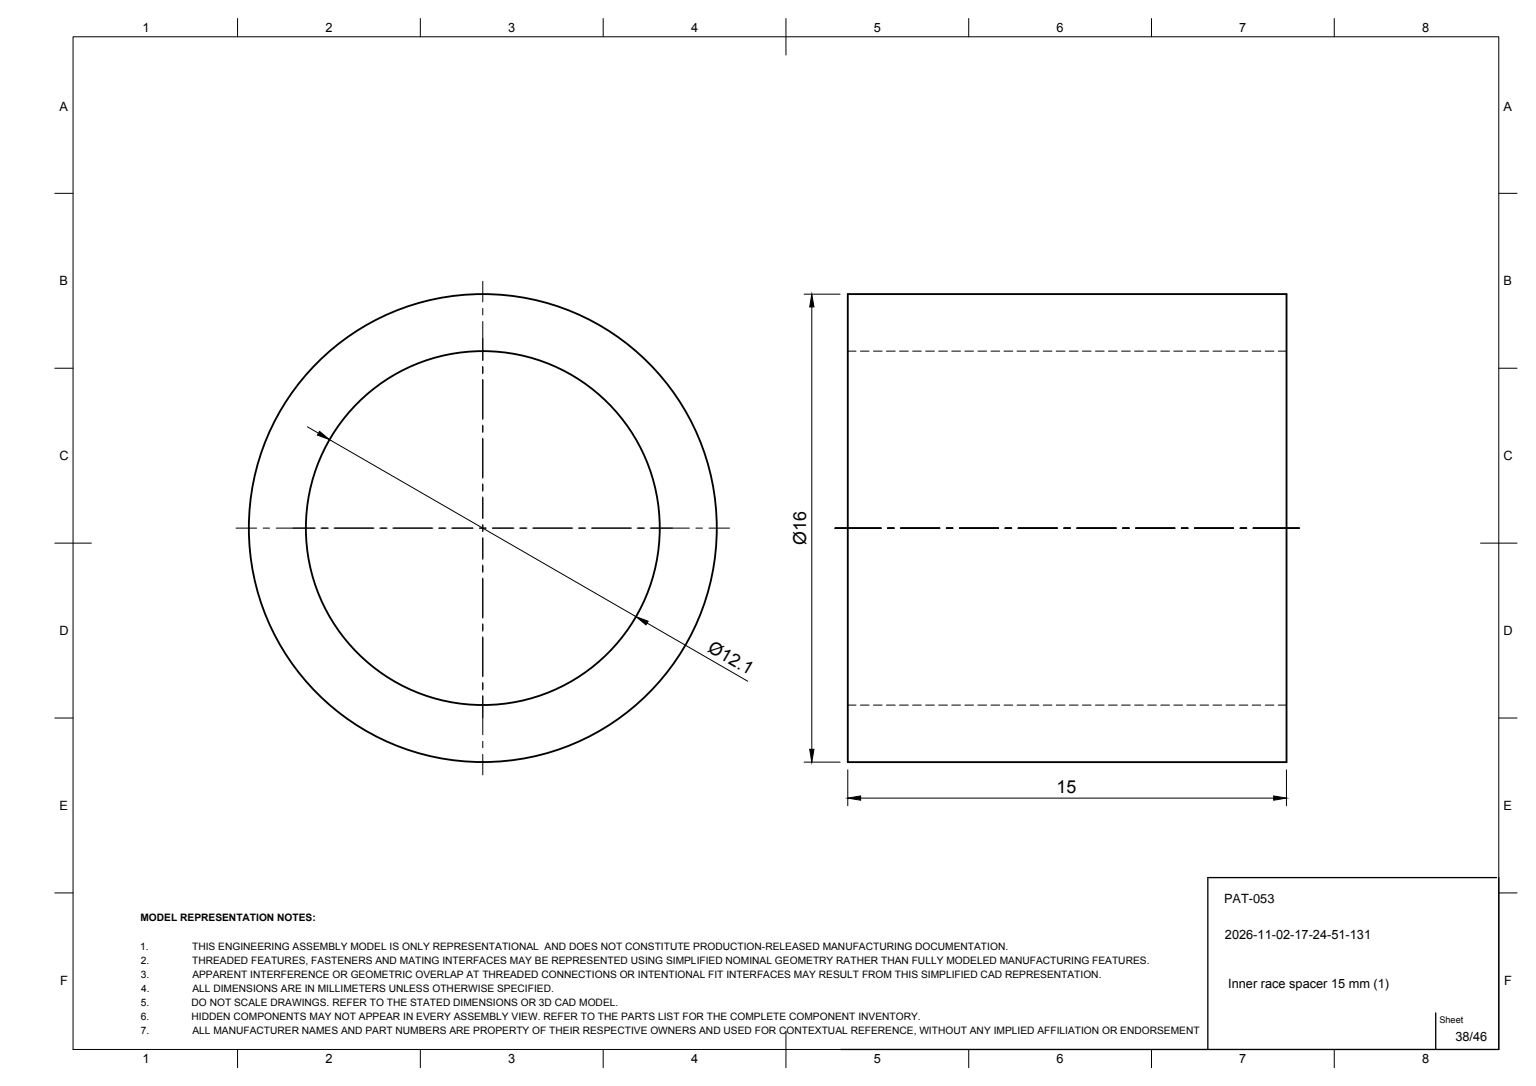
ISO-10303-21;
HEADER;
/* Generated by software containing ST-Developer
 * from STEP Tools, Inc. (www.steptools.com) 
 */

FILE_DESCRIPTION(
/* description */ ('Hand-operated arbor press'),
/* implementation_level */ '2;1');

FILE_NAME(
/* name */ 'Inner race spacer 15 mm (1).step',
/* time_stamp */ '2026-10-28T03:25:25-07:00',
/* author */ (''),
/* organization */ (''),
/* preprocessor_version */ 'ST-DEVELOPER v20.2',
/* originating_system */ 'Autodesk Translation Framework v15.17.0.0',
/* authorisation */ '');

FILE_SCHEMA (('AUTOMOTIVE_DESIGN { 1 0 10303 214 3 1 1 }'));
ENDSEC;

DATA;
#10=MECHANICAL_DESIGN_GEOMETRIC_PRESENTATION_REPRESENTATION('',(#623),#32751);
#532=SHAPE_REPRESENTATION_RELATIONSHIP('SRR','None',#32964,#574);
#574=ADVANCED_BREP_SHAPE_REPRESENTATION('',(#670),#32738);
#623=STYLED_ITEM('',(#33242),#670);
#670=MANIFOLD_SOLID_BREP('Body1',#12522);
#827=FACE_BOUND('',#2634,.T.);
#828=FACE_BOUND('',#2636,.T.);
#1212=PLANE('',#13856);
#1213=PLANE('',#13857);
#1803=FACE_OUTER_BOUND('',#2631,.T.);
#1804=FACE_OUTER_BOUND('',#2632,.T.);
#1805=FACE_OUTER_BOUND('',#2633,.T.);
#1806=FACE_OUTER_BOUND('',#2635,.T.);
#2631=EDGE_LOOP('',(#10824,#10825,#10826,#10827));
#2632=EDGE_LOOP('',(#10828,#10829,#10830,#10831));
#2633=EDGE_LOOP('',(#10832));
#2634=EDGE_LOOP('',(#10833));
#2635=EDGE_LOOP('',(#10834));
#2636=EDGE_LOOP('',(#10835));
#3760=LINE('',#20648,#4931);
#3761=LINE('',#20654,#4932);
#4931=VECTOR('',#16797,0.605);
#4932=VECTOR('',#16804,0.8);
#5462=CIRCLE('',#13851,0.605);
#5463=CIRCLE('',#13852,0.605);
#5464=CIRCLE('',#13854,0.8);
#5465=CIRCLE('',#13855,0.8);
#6395=VERTEX_POINT('',#20645);
#6396=VERTEX_POINT('',#20647);
#6397=VERTEX_POINT('',#20651);
#6398=VERTEX_POINT('',#20653);
#7915=EDGE_CURVE('',#6395,#6395,#5462,.T.);
#7916=EDGE_CURVE('',#6395,#6396,#3760,.T.);
#7917=EDGE_CURVE('',#6396,#6396,#5463,.T.);
#7918=EDGE_CURVE('',#6397,#6397,#5464,.T.);
#7919=EDGE_CURVE('',#6397,#6398,#3761,.T.);
#7920=EDGE_CURVE('',#6398,#6398,#5465,.T.);
#10824=ORIENTED_EDGE('',*,*,#7915,.F.);
#10825=ORIENTED_EDGE('',*,*,#7916,.T.);
#10826=ORIENTED_EDGE('',*,*,#7917,.T.);
#10827=ORIENTED_EDGE('',*,*,#7916,.F.);
#10828=ORIENTED_EDGE('',*,*,#7918,.F.);
#10829=ORIENTED_EDGE('',*,*,#7919,.T.);
#10830=ORIENTED_EDGE('',*,*,#7920,.T.);
#10831=ORIENTED_EDGE('',*,*,#7919,.F.);
#10832=ORIENTED_EDGE('',*,*,#7918,.T.);
#10833=ORIENTED_EDGE('',*,*,#7915,.T.);
#10834=ORIENTED_EDGE('',*,*,#7920,.F.);
#10835=ORIENTED_EDGE('',*,*,#7917,.F.);
#11760=CYLINDRICAL_SURFACE('',#13850,0.605);
#11761=CYLINDRICAL_SURFACE('',#13853,0.8);
#12312=ADVANCED_FACE('',(#1803),#11760,.F.);
#12313=ADVANCED_FACE('',(#1804),#11761,.T.);
#12314=ADVANCED_FACE('',(#1805,#827),#1212,.T.);
#12315=ADVANCED_FACE('',(#1806,#828),#1213,.F.);
#12522=CLOSED_SHELL('',(#12312,#12313,#12314,#12315));
#13849=AXIS2_PLACEMENT_3D('',#20643,#16791,#16792);
#13850=AXIS2_PLACEMENT_3D('',#20644,#16793,#16794);
#13851=AXIS2_PLACEMENT_3D('',#20646,#16795,#16796);
#13852=AXIS2_PLACEMENT_3D('',#20649,#16798,#16799);
#13853=AXIS2_PLACEMENT_3D('',#20650,#16800,#16801);
#13854=AXIS2_PLACEMENT_3D('',#20652,#16802,#16803);
#13855=AXIS2_PLACEMENT_3D('',#20655,#16805,#16806);
#13856=AXIS2_PLACEMENT_3D('',#20656,#16807,#16808);
#13857=AXIS2_PLACEMENT_3D('',#20657,#16809,#16810);
#16791=DIRECTION('axis',(0.,0.,1.));
#16792=DIRECTION('refdir',(1.,0.,0.));
#16793=DIRECTION('center_axis',(0.,1.,0.));
#16794=DIRECTION('ref_axis',(1.,0.,0.));
#16795=DIRECTION('center_axis',(0.,-1.,0.));
#16796=DIRECTION('ref_axis',(1.,0.,0.));
#16797=DIRECTION('',(0.,-1.,0.));
#16798=DIRECTION('center_axis',(0.,-1.,0.));
#16799=DIRECTION('ref_axis',(1.,0.,0.));
#16800=DIRECTION('center_axis',(0.,1.,0.));
#16801=DIRECTION('ref_axis',(1.,0.,0.));
#16802=DIRECTION('center_axis',(0.,1.,0.));
#16803=DIRECTION('ref_axis',(1.,0.,0.));
#16804=DIRECTION('',(0.,-1.,0.));
#16805=DIRECTION('center_axis',(0.,1.,0.));
#16806=DIRECTION('ref_axis',(1.,0.,0.));
#16807=DIRECTION('center_axis',(0.,1.,0.));
#16808=DIRECTION('ref_axis',(1.,0.,0.));
#16809=DIRECTION('center_axis',(0.,1.,0.));
#16810=DIRECTION('ref_axis',(1.,0.,0.));
#20643=CARTESIAN_POINT('',(0.,0.,0.));
#20644=CARTESIAN_POINT('Origin',(-3.25,3.5,20.));
#20645=CARTESIAN_POINT('',(-3.855,5.,20.));
#20646=CARTESIAN_POINT('Origin',(-3.25,5.,20.));
#20647=CARTESIAN_POINT('',(-3.855,3.5,20.));
#20648=CARTESIAN_POINT('',(-3.855,3.5,20.));
#20649=CARTESIAN_POINT('Origin',(-3.25,3.5,20.));
#20650=CARTESIAN_POINT('Origin',(-3.25,3.5,20.));
#20651=CARTESIAN_POINT('',(-4.05,5.,20.));
#20652=CARTESIAN_POINT('Origin',(-3.25,5.,20.));
#20653=CARTESIAN_POINT('',(-4.05,3.5,20.));
#20654=CARTESIAN_POINT('',(-4.05,3.5,20.));
#20655=CARTESIAN_POINT('Origin',(-3.25,3.5,20.));
#20656=CARTESIAN_POINT('Origin',(-3.25,5.,20.));
#20657=CARTESIAN_POINT('Origin',(-3.25,3.5,20.));
#32689=UNCERTAINTY_MEASURE_WITH_UNIT(LENGTH_MEASURE(0.001),#32752,
'DISTANCE_ACCURACY_VALUE',
'Maximum model space distance between geometric entities at asserted c
onnectivities');
#32702=UNCERTAINTY_MEASURE_WITH_UNIT(LENGTH_MEASURE(0.001),#32752,
'DISTANCE_ACCURACY_VALUE',
'Maximum model space distance between geometric entities at asserted c
onnectivities');
#32738=(
GEOMETRIC_REPRESENTATION_CONTEXT(3)
GLOBAL_UNCERTAINTY_ASSIGNED_CONTEXT((#32689))
GLOBAL_UNIT_ASSIGNED_CONTEXT((#32752,#32754,#32755))
REPRESENTATION_CONTEXT('','3D')
);
#32751=(
GEOMETRIC_REPRESENTATION_CONTEXT(3)
GLOBAL_UNCERTAINTY_ASSIGNED_CONTEXT((#32702))
GLOBAL_UNIT_ASSIGNED_CONTEXT((#32752,#32754,#32755))
REPRESENTATION_CONTEXT('','3D')
);
#32752=(
LENGTH_UNIT()
NAMED_UNIT(*)
SI_UNIT(.CENTI.,.METRE.)
);
#32754=(
NAMED_UNIT(*)
PLANE_ANGLE_UNIT()
SI_UNIT($,.RADIAN.)
);
#32755=(
NAMED_UNIT(*)
SI_UNIT($,.STERADIAN.)
SOLID_ANGLE_UNIT()
);
#32791=SHAPE_DEFINITION_REPRESENTATION(#32848,#32964);
#32848=PRODUCT_DEFINITION_SHAPE('',$,#33013);
#32964=SHAPE_REPRESENTATION('',(#13849),#32738);
#32977=PRODUCT_DEFINITION_CONTEXT('part definition',#33123,'design');
#33013=PRODUCT_DEFINITION('Inner race spacer 15 mm (1)',
'Inner race spacer 15 mm (1)',#33061,#32977);
#33061=PRODUCT_DEFINITION_FORMATION('',$,#33160);
#33123=APPLICATION_CONTEXT(
'Core Data for Automotive Mechanical Design Process');
#33124=PRODUCT_CONTEXT('part definition',#33123,'mechanical');
#33160=PRODUCT('Inner race spacer 15 mm (1)',
'Inner race spacer 15 mm (1)','Inner race spacer 15 mm (1)',(#33124));
#33236=COLOUR_RGB('Grey',0.48,0.52,0.57);
#33237=FILL_AREA_STYLE_COLOUR('',#33236);
#33238=FILL_AREA_STYLE('',(#33237));
#33239=SURFACE_STYLE_FILL_AREA(#33238);
#33240=SURFACE_SIDE_STYLE('',(#33239));
#33241=SURFACE_STYLE_USAGE(.BOTH.,#33240);
#33242=PRESENTATION_STYLE_ASSIGNMENT((#33241));
ENDSEC;
END-ISO-10303-21;
